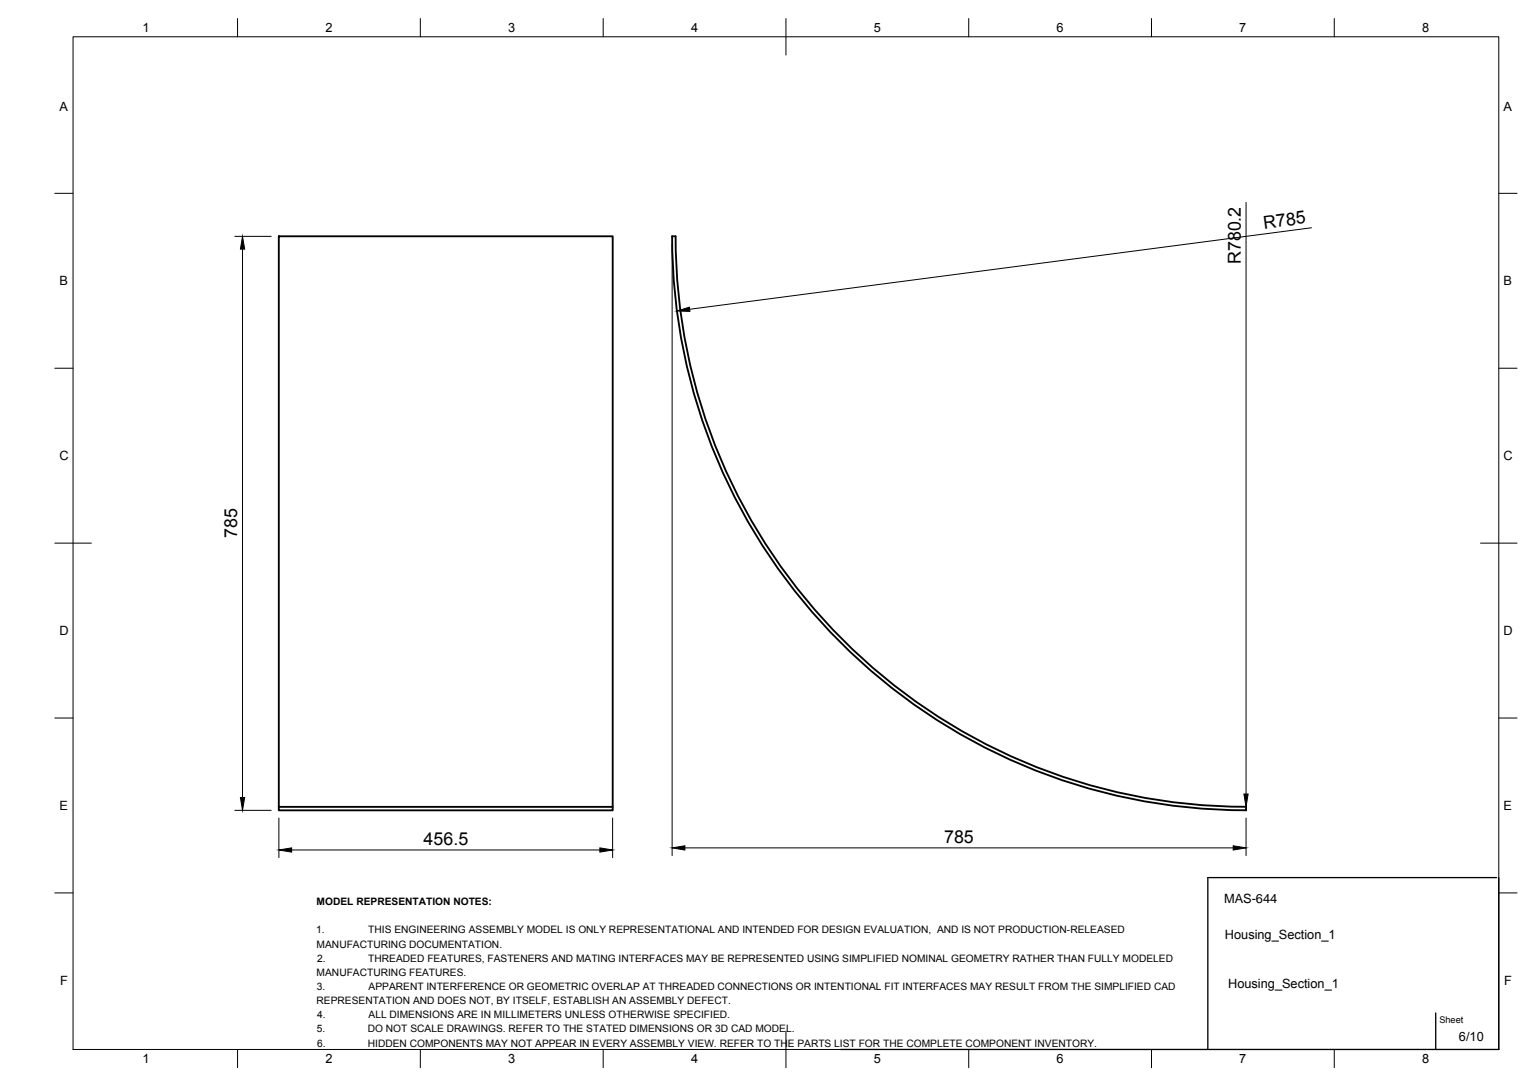
ISO-10303-21;
HEADER;
FILE_DESCRIPTION((''),'2;1');
FILE_NAME('Housing_Section_1.step','2026-10-09T11:38:21-07:00',(''),(''),'','','');
FILE_SCHEMA (('AUTOMOTIVE_DESIGN { 1 0 10303 214 3 1 1 }'));
ENDSEC;
DATA;
#10=MECHANICAL_DESIGN_GEOMETRIC_PRESENTATION_REPRESENTATION('',(#62),#3619);
#46=SHAPE_REPRESENTATION_RELATIONSHIP('SRR','None',#3654,#54) ;
#54=ADVANCED_BREP_SHAPE_REPRESENTATION('',(#70),#3614) ;
#62=STYLED_ITEM('',(#3700),#70) ;
#70=MANIFOLD_SOLID_BREP('Body1',#2086) ;
#183=PLANE('',#2346) ;
#184=PLANE('',#2350) ;
#185=PLANE('',#2351) ;
#186=PLANE('',#2352) ;
#283=FACE_OUTER_BOUND('',#473,.T.) ;
#284=FACE_OUTER_BOUND('',#474,.T.) ;
#285=FACE_OUTER_BOUND('',#475,.T.) ;
#286=FACE_OUTER_BOUND('',#476,.T.) ;
#287=FACE_OUTER_BOUND('',#477,.T.) ;
#288=FACE_OUTER_BOUND('',#478,.T.) ;
#473=EDGE_LOOP('',(#1771,#1772,#1773,#1774)) ;
#474=EDGE_LOOP('',(#1775,#1776,#1777,#1778)) ;
#475=EDGE_LOOP('',(#1779,#1780,#1781,#1782)) ;
#476=EDGE_LOOP('',(#1783,#1784,#1785,#1786)) ;
#477=EDGE_LOOP('',(#1787,#1788,#1789,#1790)) ;
#478=EDGE_LOOP('',(#1791,#1792,#1793,#1794)) ;
#615=LINE('',#3431,#779) ;
#616=LINE('',#3434,#780) ;
#617=LINE('',#3437,#781) ;
#618=LINE('',#3439,#782) ;
#619=LINE('',#3440,#783) ;
#620=LINE('',#3445,#784) ;
#621=LINE('',#3448,#785) ;
#622=LINE('',#3449,#786) ;
#779=VECTOR('',#2843,1000.) ;
#780=VECTOR('',#2846,1000.) ;
#781=VECTOR('',#2849,1000.) ;
#782=VECTOR('',#2850,1000.) ;
#783=VECTOR('',#2851,1000.) ;
#784=VECTOR('',#2856,1000.) ;
#785=VECTOR('',#2861,1000.) ;
#786=VECTOR('',#2862,1000.) ;
#927=CIRCLE('',#2344,780.2) ;
#928=CIRCLE('',#2345,780.2) ;
#929=CIRCLE('',#2348,785.) ;
#930=CIRCLE('',#2349,785.) ;
#1071=VERTEX_POINT('',#3427) ;
#1072=VERTEX_POINT('',#3428) ;
#1073=VERTEX_POINT('',#3430) ;
#1074=VERTEX_POINT('',#3432) ;
#1075=VERTEX_POINT('',#3436) ;
#1076=VERTEX_POINT('',#3438) ;
#1077=VERTEX_POINT('',#3442) ;
#1078=VERTEX_POINT('',#3444) ;
#1311=EDGE_CURVE('',#1071,#1072,#927,.T.) ;
#1312=EDGE_CURVE('',#1073,#1072,#615,.T.) ;
#1313=EDGE_CURVE('',#1074,#1073,#928,.T.) ;
#1314=EDGE_CURVE('',#1074,#1071,#616,.T.) ;
#1315=EDGE_CURVE('',#1075,#1072,#617,.T.) ;
#1316=EDGE_CURVE('',#1076,#1075,#618,.T.) ;
#1317=EDGE_CURVE('',#1076,#1073,#619,.T.) ;
#1318=EDGE_CURVE('',#1077,#1075,#929,.T.) ;
#1319=EDGE_CURVE('',#1078,#1077,#620,.T.) ;
#1320=EDGE_CURVE('',#1078,#1076,#930,.T.) ;
#1321=EDGE_CURVE('',#1071,#1077,#621,.T.) ;
#1322=EDGE_CURVE('',#1074,#1078,#622,.T.) ;
#1771=ORIENTED_EDGE('',*,*,#1311,.T.) ;
#1772=ORIENTED_EDGE('',*,*,#1312,.F.) ;
#1773=ORIENTED_EDGE('',*,*,#1313,.F.) ;
#1774=ORIENTED_EDGE('',*,*,#1314,.T.) ;
#1775=ORIENTED_EDGE('',*,*,#1315,.F.) ;
#1776=ORIENTED_EDGE('',*,*,#1316,.F.) ;
#1777=ORIENTED_EDGE('',*,*,#1317,.T.) ;
#1778=ORIENTED_EDGE('',*,*,#1312,.T.) ;
#1779=ORIENTED_EDGE('',*,*,#1318,.F.) ;
#1780=ORIENTED_EDGE('',*,*,#1319,.F.) ;
#1781=ORIENTED_EDGE('',*,*,#1320,.T.) ;
#1782=ORIENTED_EDGE('',*,*,#1316,.T.) ;
#1783=ORIENTED_EDGE('',*,*,#1321,.F.) ;
#1784=ORIENTED_EDGE('',*,*,#1314,.F.) ;
#1785=ORIENTED_EDGE('',*,*,#1322,.T.) ;
#1786=ORIENTED_EDGE('',*,*,#1319,.T.) ;
#1787=ORIENTED_EDGE('',*,*,#1313,.T.) ;
#1788=ORIENTED_EDGE('',*,*,#1317,.F.) ;
#1789=ORIENTED_EDGE('',*,*,#1320,.F.) ;
#1790=ORIENTED_EDGE('',*,*,#1322,.F.) ;
#1791=ORIENTED_EDGE('',*,*,#1311,.F.) ;
#1792=ORIENTED_EDGE('',*,*,#1321,.T.) ;
#1793=ORIENTED_EDGE('',*,*,#1318,.T.) ;
#1794=ORIENTED_EDGE('',*,*,#1315,.T.) ;
#1967=CYLINDRICAL_SURFACE('',#2343,780.2) ;
#1968=CYLINDRICAL_SURFACE('',#2347,785.) ;
#2045=ADVANCED_FACE('',(#283),#1967,.F.) ;
#2046=ADVANCED_FACE('',(#284),#183,.T.) ;
#2047=ADVANCED_FACE('',(#285),#1968,.T.) ;
#2048=ADVANCED_FACE('',(#286),#184,.T.) ;
#2049=ADVANCED_FACE('',(#287),#185,.T.) ;
#2050=ADVANCED_FACE('',(#288),#186,.F.) ;
#2086=CLOSED_SHELL('',(#2045,#2046,#2047,#2048,#2049,#2050)) ;
#2342=AXIS2_PLACEMENT_3D('',#3425,#2837,#2838) ;
#2343=AXIS2_PLACEMENT_3D('',#3426,#2839,#2840) ;
#2344=AXIS2_PLACEMENT_3D('',#3429,#2841,#2842) ;
#2345=AXIS2_PLACEMENT_3D('',#3433,#2844,#2845) ;
#2346=AXIS2_PLACEMENT_3D('',#3435,#2847,#2848) ;
#2347=AXIS2_PLACEMENT_3D('',#3441,#2852,#2853) ;
#2348=AXIS2_PLACEMENT_3D('',#3443,#2854,#2855) ;
#2349=AXIS2_PLACEMENT_3D('',#3446,#2857,#2858) ;
#2350=AXIS2_PLACEMENT_3D('',#3447,#2859,#2860) ;
#2351=AXIS2_PLACEMENT_3D('',#3450,#2863,#2864) ;
#2352=AXIS2_PLACEMENT_3D('',#3451,#2865,#2866) ;
#2837=DIRECTION('axis',(0.,0.,1.)) ;
#2838=DIRECTION('refdir',(1.,0.,0.)) ;
#2839=DIRECTION('center_axis',(0.,0.,-1.)) ;
#2840=DIRECTION('ref_axis',(-1.,0.,0.)) ;
#2841=DIRECTION('center_axis',(0.,0.,-1.)) ;
#2842=DIRECTION('ref_axis',(1.,0.,0.)) ;
#2843=DIRECTION('',(0.,0.,-1.)) ;
#2844=DIRECTION('center_axis',(0.,0.,-1.)) ;
#2845=DIRECTION('ref_axis',(1.,0.,0.)) ;
#2846=DIRECTION('',(0.,0.,-1.)) ;
#2847=DIRECTION('center_axis',(-1.,-5.99005365632946E-14,0.)) ;
#2848=DIRECTION('ref_axis',(5.99005365632946E-14,-1.,0.)) ;
#2849=DIRECTION('',(-5.99005365632946E-14,1.,0.)) ;
#2850=DIRECTION('',(0.,0.,-1.)) ;
#2851=DIRECTION('',(-5.99005365632946E-14,1.,0.)) ;
#2852=DIRECTION('center_axis',(0.,0.,-1.)) ;
#2853=DIRECTION('ref_axis',(-1.,0.,0.)) ;
#2854=DIRECTION('center_axis',(0.,0.,-1.)) ;
#2855=DIRECTION('ref_axis',(-1.,0.,0.)) ;
#2856=DIRECTION('',(0.,0.,-1.)) ;
#2857=DIRECTION('center_axis',(0.,0.,-1.)) ;
#2858=DIRECTION('ref_axis',(-1.,0.,0.)) ;
#2859=DIRECTION('center_axis',(-1.22464679914736E-16,1.,0.)) ;
#2860=DIRECTION('ref_axis',(-1.,-1.22464679914736E-16,0.)) ;
#2861=DIRECTION('',(1.,1.22464679914736E-16,0.)) ;
#2862=DIRECTION('',(1.,1.22464679914736E-16,0.)) ;
#2863=DIRECTION('center_axis',(0.,0.,1.)) ;
#2864=DIRECTION('ref_axis',(1.,0.,0.)) ;
#2865=DIRECTION('center_axis',(0.,0.,1.)) ;
#2866=DIRECTION('ref_axis',(1.,0.,0.)) ;
#3425=CARTESIAN_POINT('',(0.,0.,0.)) ;
#3426=CARTESIAN_POINT('Origin',(99.9999999999999,1.35813926733553E-13,456.5)) ;
#3427=CARTESIAN_POINT('',(880.2,2.3136087000303E-13,-5.55111512312578E-14)) ;
#3428=CARTESIAN_POINT('',(99.9999999999997,-780.2,-5.55111512312578E-14)) ;
#3429=CARTESIAN_POINT('Origin',(99.9999999999999,1.35813926733553E-13,-5.55111512312578E-14)) ;
#3430=CARTESIAN_POINT('',(99.9999999999997,-780.2,456.5)) ;
#3431=CARTESIAN_POINT('',(99.9999999999997,-780.2,456.5)) ;
#3432=CARTESIAN_POINT('',(880.2,2.3136087000303E-13,456.5)) ;
#3433=CARTESIAN_POINT('Origin',(99.9999999999999,1.35813926733553E-13,456.5)) ;
#3434=CARTESIAN_POINT('',(880.2,2.3136087000303E-13,456.5)) ;
#3435=CARTESIAN_POINT('Origin',(100.,-785.,456.5)) ;
#3436=CARTESIAN_POINT('',(100.,-785.,-5.55111512312578E-14)) ;
#3437=CARTESIAN_POINT('',(100.,-785.,-5.55111512312578E-14)) ;
#3438=CARTESIAN_POINT('',(100.,-785.,456.5)) ;
#3439=CARTESIAN_POINT('',(100.,-785.,456.5)) ;
#3440=CARTESIAN_POINT('',(100.,-785.,456.5)) ;
#3441=CARTESIAN_POINT('Origin',(99.9999999999999,1.35813926733553E-13,456.5)) ;
#3442=CARTESIAN_POINT('',(885.,2.3194870046662E-13,-5.55111512312578E-14)) ;
#3443=CARTESIAN_POINT('Origin',(99.9999999999999,1.35813926733553E-13,-5.55111512312578E-14)) ;
#3444=CARTESIAN_POINT('',(885.,2.3194870046662E-13,456.5)) ;
#3445=CARTESIAN_POINT('',(885.,2.3194870046662E-13,456.5)) ;
#3446=CARTESIAN_POINT('Origin',(99.9999999999999,1.35813926733553E-13,456.5)) ;
#3447=CARTESIAN_POINT('Origin',(880.2,2.3136087000303E-13,456.5)) ;
#3448=CARTESIAN_POINT('',(880.2,2.3136087000303E-13,-5.55111512312578E-14)) ;
#3449=CARTESIAN_POINT('',(880.2,2.3136087000303E-13,456.5)) ;
#3450=CARTESIAN_POINT('Origin',(99.9999999999999,1.35813926733553E-13,456.5)) ;
#3451=CARTESIAN_POINT('Origin',(99.9999999999999,1.35813926733553E-13,-5.55111512312578E-14)) ;
#3604=UNCERTAINTY_MEASURE_WITH_UNIT(LENGTH_MEASURE(0.01),#3620,
'DISTANCE_ACCURACY_VALUE',
'Maximum model space distance between geometric entities at asserted c
onnectivities') ;
#3609=UNCERTAINTY_MEASURE_WITH_UNIT(LENGTH_MEASURE(0.01),#3620,
'DISTANCE_ACCURACY_VALUE',
'Maximum model space distance between geometric entities at asserted c
onnectivities') ;
#3614=(
GEOMETRIC_REPRESENTATION_CONTEXT(3)
GLOBAL_UNCERTAINTY_ASSIGNED_CONTEXT((#3604))
GLOBAL_UNIT_ASSIGNED_CONTEXT((#3620,#3622,#3623))
REPRESENTATION_CONTEXT('','3D')
) ;
#3619=(
GEOMETRIC_REPRESENTATION_CONTEXT(3)
GLOBAL_UNCERTAINTY_ASSIGNED_CONTEXT((#3609))
GLOBAL_UNIT_ASSIGNED_CONTEXT((#3620,#3622,#3623))
REPRESENTATION_CONTEXT('','3D')
) ;
#3620=(
LENGTH_UNIT()
NAMED_UNIT(*)
SI_UNIT(.MILLI.,.METRE.)
) ;
#3622=(
NAMED_UNIT(*)
PLANE_ANGLE_UNIT()
SI_UNIT($,.RADIAN.)
) ;
#3623=(
NAMED_UNIT(*)
SI_UNIT($,.STERADIAN.)
SOLID_ANGLE_UNIT()
) ;
#3628=SHAPE_DEFINITION_REPRESENTATION(#3637,#3654) ;
#3637=PRODUCT_DEFINITION_SHAPE('',$,#3664) ;
#3654=SHAPE_REPRESENTATION('',(#2342),#3614) ;
#3659=PRODUCT_DEFINITION_CONTEXT('part definition',#3688,'design') ;
#3664=PRODUCT_DEFINITION('Housing_Section_1','Housing_Section_1',#3673,
#3659) ;
#3673=PRODUCT_DEFINITION_FORMATION('',$,#3694) ;
#3688=APPLICATION_CONTEXT(
'Core Data for Automotive Mechanical Design Process') ;
#3689=PRODUCT_CONTEXT('part definition',#3688,'mechanical') ;
#3694=PRODUCT('Housing_Section_1','Housing_Section_1',$,(#3689)) ;
#3700=PRESENTATION_STYLE_ASSIGNMENT((#3702)) ;
#3702=SURFACE_STYLE_USAGE(.BOTH.,#3704) ;
#3704=SURFACE_SIDE_STYLE('',(#3706)) ;
#3706=SURFACE_STYLE_FILL_AREA(#3708) ;
#3708=FILL_AREA_STYLE('Opaque(202,209,238)',(#3710)) ;
#3710=FILL_AREA_STYLE_COLOUR('Opaque(202,209,238)',#3712) ;
#3712=COLOUR_RGB('Opaque(202,209,238)', 0.09019608, 0.27058824, 0.51372549) ;
ENDSEC;
END-ISO-10303-21;
